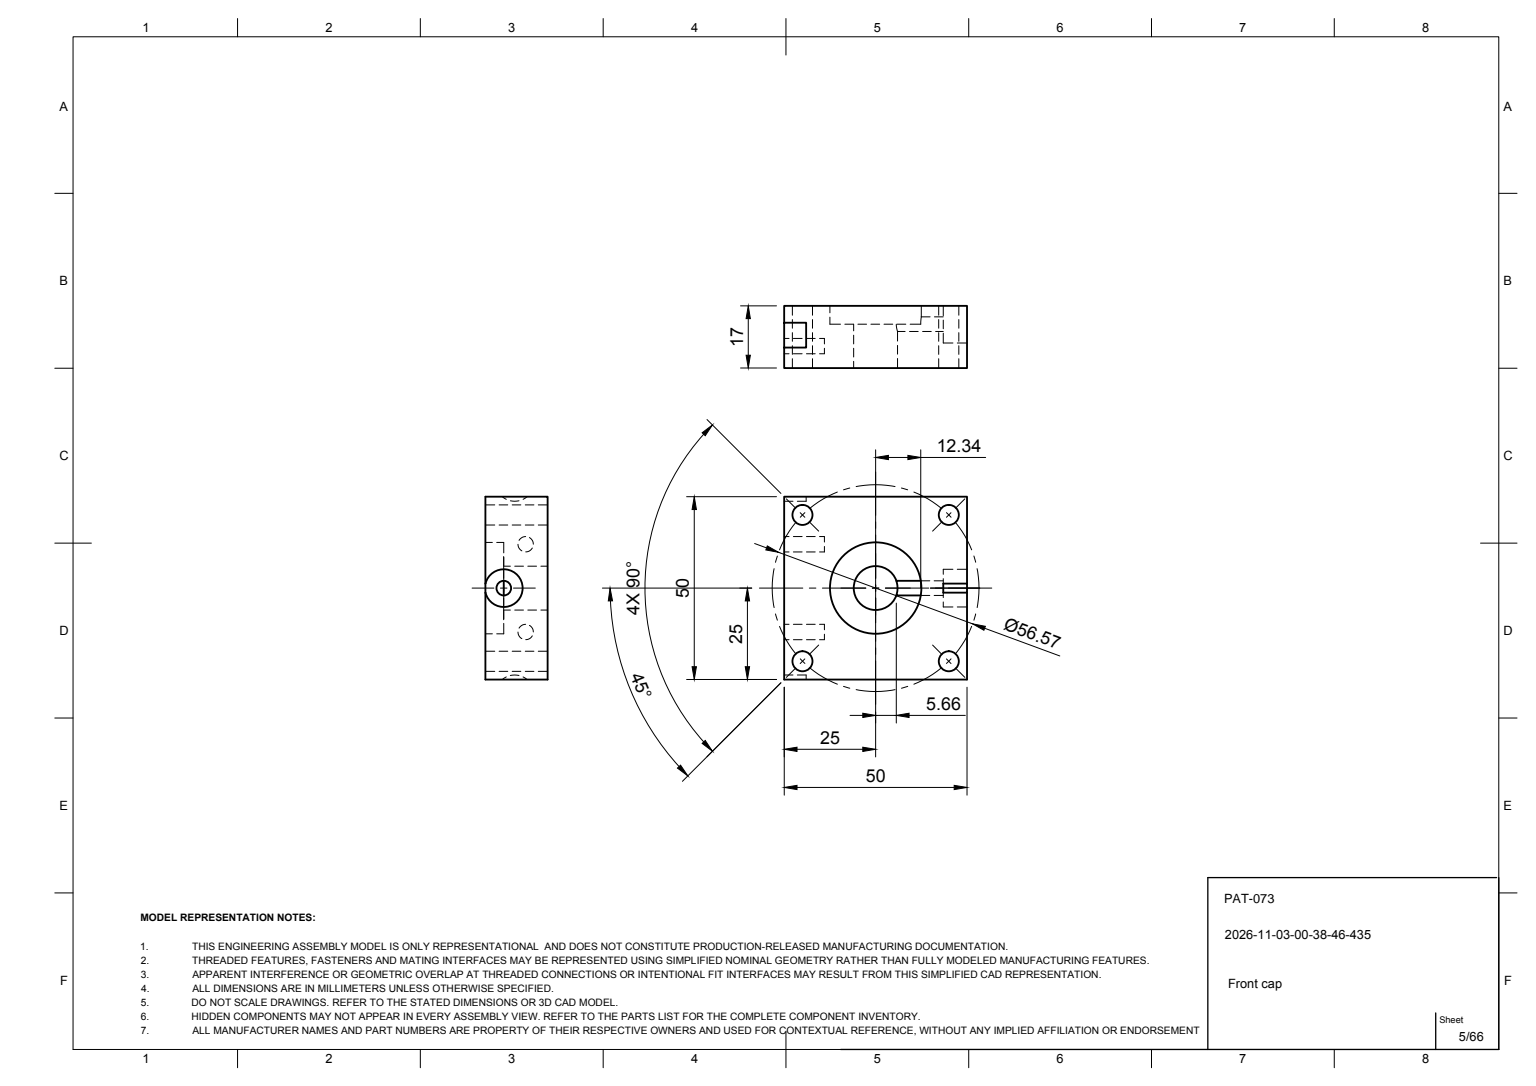
ISO-10303-21;
HEADER;
/* Generated by software containing ST-Developer
 * from STEP Tools, Inc. (www.steptools.com) 
 */

FILE_DESCRIPTION(
/* description */ ('Manual piston pump'),
/* implementation_level */ '2;1');

FILE_NAME(
/* name */ 'Front cap.step',
/* time_stamp */ '2026-11-02T16:54:23-08:00',
/* author */ (''),
/* organization */ (''),
/* preprocessor_version */ 'ST-DEVELOPER v20.2',
/* originating_system */ 'Autodesk Translation Framework v15.17.0.0',
/* authorisation */ '');

FILE_SCHEMA (('AUTOMOTIVE_DESIGN { 1 0 10303 214 3 1 1 }'));
ENDSEC;

DATA;
#10=MECHANICAL_DESIGN_GEOMETRIC_PRESENTATION_REPRESENTATION('',(#688),#19043);
#562=SHAPE_REPRESENTATION_RELATIONSHIP('SRR','None',#19308,#625);
#625=ADVANCED_BREP_SHAPE_REPRESENTATION('',(#760),#18975);
#688=STYLED_ITEM('',(#19661),#760);
#760=MANIFOLD_SOLID_BREP('Body1',#9472);
#827=FACE_BOUND('',#1879,.T.);
#828=FACE_BOUND('',#1882,.T.);
#829=FACE_BOUND('',#1883,.T.);
#830=FACE_BOUND('',#1884,.T.);
#831=FACE_BOUND('',#1885,.T.);
#832=FACE_BOUND('',#1886,.T.);
#833=FACE_BOUND('',#1895,.T.);
#834=FACE_BOUND('',#1896,.T.);
#835=FACE_BOUND('',#1897,.T.);
#836=FACE_BOUND('',#1898,.T.);
#837=FACE_BOUND('',#1899,.T.);
#838=FACE_BOUND('',#1902,.T.);
#839=FACE_BOUND('',#1903,.T.);
#1048=B_SPLINE_CURVE_WITH_KNOTS('',3,(#14655,#14656,#14657,#14658,#14659,
#14660,#14661,#14662,#14663,#14664,#14665,#14666,#14667,#14668,#14669,#14670,
#14671,#14672),.UNSPECIFIED.,.F.,.F.,(4,2,2,2,2,2,2,2,4),(0.,0.0754777383366878,
0.150955476673376,0.226431506332747,0.301907535992118,0.377383565651489,
0.45285959531086,0.528337333647548,0.603815071984236),.UNSPECIFIED.);
#1049=B_SPLINE_CURVE_WITH_KNOTS('',3,(#14676,#14677,#14678,#14679,#14680,
#14681,#14682,#14683,#14684,#14685,#14686,#14687,#14688,#14689,#14690,#14691,
#14692,#14693),.UNSPECIFIED.,.F.,.F.,(4,2,2,2,2,2,2,2,4),(-0.607760117460593,
-0.531772481215855,-0.455784844971118,-0.379832451850707,-0.303880058730296,
-0.227927665609885,-0.151975272489475,-0.0759876362447374,0.),
 .UNSPECIFIED.);
#1091=CYLINDRICAL_SURFACE('',#10248,0.525);
#1092=CYLINDRICAL_SURFACE('',#10250,0.525);
#1093=CYLINDRICAL_SURFACE('',#10255,0.21);
#1094=CYLINDRICAL_SURFACE('',#10259,0.21);
#1095=CYLINDRICAL_SURFACE('',#10263,0.2);
#1096=CYLINDRICAL_SURFACE('',#10265,0.6);
#1097=CYLINDRICAL_SURFACE('',#10271,0.515);
#1098=CYLINDRICAL_SURFACE('',#10279,0.275);
#1099=CYLINDRICAL_SURFACE('',#10281,0.275);
#1100=CYLINDRICAL_SURFACE('',#10283,0.275);
#1101=CYLINDRICAL_SURFACE('',#10285,0.275);
#1102=CYLINDRICAL_SURFACE('',#10287,1.25);
#1292=FACE_OUTER_BOUND('',#1867,.T.);
#1293=FACE_OUTER_BOUND('',#1868,.T.);
#1294=FACE_OUTER_BOUND('',#1869,.T.);
#1295=FACE_OUTER_BOUND('',#1870,.T.);
#1296=FACE_OUTER_BOUND('',#1871,.T.);
#1297=FACE_OUTER_BOUND('',#1872,.T.);
#1298=FACE_OUTER_BOUND('',#1873,.T.);
#1299=FACE_OUTER_BOUND('',#1874,.T.);
#1300=FACE_OUTER_BOUND('',#1875,.T.);
#1301=FACE_OUTER_BOUND('',#1876,.T.);
#1302=FACE_OUTER_BOUND('',#1877,.T.);
#1303=FACE_OUTER_BOUND('',#1878,.T.);
#1304=FACE_OUTER_BOUND('',#1880,.T.);
#1305=FACE_OUTER_BOUND('',#1881,.T.);
#1306=FACE_OUTER_BOUND('',#1887,.T.);
#1307=FACE_OUTER_BOUND('',#1888,.T.);
#1308=FACE_OUTER_BOUND('',#1889,.T.);
#1309=FACE_OUTER_BOUND('',#1890,.T.);
#1310=FACE_OUTER_BOUND('',#1891,.T.);
#1311=FACE_OUTER_BOUND('',#1892,.T.);
#1312=FACE_OUTER_BOUND('',#1893,.T.);
#1313=FACE_OUTER_BOUND('',#1894,.T.);
#1314=FACE_OUTER_BOUND('',#1900,.T.);
#1315=FACE_OUTER_BOUND('',#1901,.T.);
#1867=EDGE_LOOP('',(#6273,#6274));
#1868=EDGE_LOOP('',(#6275,#6276,#6277,#6278));
#1869=EDGE_LOOP('',(#6279,#6280,#6281,#6282));
#1870=EDGE_LOOP('',(#6283,#6284));
#1871=EDGE_LOOP('',(#6285,#6286,#6287,#6288,#6289,#6290,#6291,#6292));
#1872=EDGE_LOOP('',(#6293,#6294,#6295,#6296));
#1873=EDGE_LOOP('',(#6297));
#1874=EDGE_LOOP('',(#6298,#6299,#6300,#6301));
#1875=EDGE_LOOP('',(#6302));
#1876=EDGE_LOOP('',(#6303,#6304,#6305,#6306,#6307,#6308,#6309));
#1877=EDGE_LOOP('',(#6310,#6311,#6312,#6313,#6314,#6315));
#1878=EDGE_LOOP('',(#6316,#6317));
#1879=EDGE_LOOP('',(#6318));
#1880=EDGE_LOOP('',(#6319,#6320,#6321,#6322));
#1881=EDGE_LOOP('',(#6323,#6324,#6325,#6326,#6327,#6328,#6329,#6330));
#1882=EDGE_LOOP('',(#6331));
#1883=EDGE_LOOP('',(#6332));
#1884=EDGE_LOOP('',(#6333));
#1885=EDGE_LOOP('',(#6334));
#1886=EDGE_LOOP('',(#6335));
#1887=EDGE_LOOP('',(#6336,#6337,#6338,#6339));
#1888=EDGE_LOOP('',(#6340,#6341,#6342,#6343));
#1889=EDGE_LOOP('',(#6344,#6345,#6346,#6347));
#1890=EDGE_LOOP('',(#6348,#6349,#6350,#6351));
#1891=EDGE_LOOP('',(#6352,#6353,#6354,#6355,#6356,#6357));
#1892=EDGE_LOOP('',(#6358,#6359,#6360,#6361,#6362,#6363));
#1893=EDGE_LOOP('',(#6364,#6365,#6366,#6367,#6368,#6369,#6370,#6371));
#1894=EDGE_LOOP('',(#6372,#6373,#6374,#6375));
#1895=EDGE_LOOP('',(#6376));
#1896=EDGE_LOOP('',(#6377));
#1897=EDGE_LOOP('',(#6378));
#1898=EDGE_LOOP('',(#6379));
#1899=EDGE_LOOP('',(#6380));
#1900=EDGE_LOOP('',(#6381,#6382,#6383,#6384,#6385,#6386));
#1901=EDGE_LOOP('',(#6387,#6388,#6389,#6390,#6391,#6392,#6393,#6394));
#1902=EDGE_LOOP('',(#6395));
#1903=EDGE_LOOP('',(#6396));
#2663=CIRCLE('',#10247,0.525);
#2664=CIRCLE('',#10249,0.525);
#2665=CIRCLE('',#10251,0.525);
#2666=CIRCLE('',#10252,0.525);
#2667=CIRCLE('',#10256,0.21);
#2668=CIRCLE('',#10257,0.21);
#2669=CIRCLE('',#10260,0.21);
#2670=CIRCLE('',#10261,0.21);
#2671=CIRCLE('',#10264,0.2);
#2672=CIRCLE('',#10266,0.6);
#2673=CIRCLE('',#10267,0.6);
#2674=CIRCLE('',#10268,0.6);
#2675=CIRCLE('',#10270,0.515);
#2676=CIRCLE('',#10272,0.515);
#2677=CIRCLE('',#10274,0.275);
#2678=CIRCLE('',#10275,0.275);
#2679=CIRCLE('',#10276,0.275);
#2680=CIRCLE('',#10277,0.275);
#2681=CIRCLE('',#10278,1.25);
#2682=CIRCLE('',#10280,0.275);
#2683=CIRCLE('',#10282,0.275);
#2684=CIRCLE('',#10284,0.275);
#2685=CIRCLE('',#10286,0.275);
#2686=CIRCLE('',#10288,1.25);
#2687=CIRCLE('',#10289,1.25);
#3147=LINE('',#14609,#3751);
#3148=LINE('',#14613,#3752);
#3149=LINE('',#14616,#3753);
#3150=LINE('',#14620,#3754);
#3151=LINE('',#14624,#3755);
#3152=LINE('',#14627,#3756);
#3153=LINE('',#14630,#3757);
#3154=LINE('',#14632,#3758);
#3155=LINE('',#14634,#3759);
#3156=LINE('',#14636,#3760);
#3157=LINE('',#14637,#3761);
#3158=LINE('',#14642,#3762);
#3159=LINE('',#14649,#3763);
#3160=LINE('',#14674,#3764);
#3161=LINE('',#14694,#3765);
#3162=LINE('',#14696,#3766);
#3163=LINE('',#14702,#3767);
#3164=LINE('',#14708,#3768);
#3165=LINE('',#14712,#3769);
#3166=LINE('',#14715,#3770);
#3167=LINE('',#14718,#3771);
#3168=LINE('',#14720,#3772);
#3169=LINE('',#14721,#3773);
#3170=LINE('',#14722,#3774);
#3171=LINE('',#14736,#3775);
#3172=LINE('',#14740,#3776);
#3173=LINE('',#14744,#3777);
#3174=LINE('',#14748,#3778);
#3175=LINE('',#14752,#3779);
#3176=LINE('',#14756,#3780);
#3177=LINE('',#14758,#3781);
#3178=LINE('',#14760,#3782);
#3179=LINE('',#14761,#3783);
#3180=LINE('',#14763,#3784);
#3181=LINE('',#14764,#3785);
#3751=VECTOR('',#11503,1.);
#3752=VECTOR('',#11508,1.);
#3753=VECTOR('',#11511,1.);
#3754=VECTOR('',#11514,1.);
#3755=VECTOR('',#11517,1.);
#3756=VECTOR('',#11522,1.);
#3757=VECTOR('',#11525,1.);
#3758=VECTOR('',#11526,1.);
#3759=VECTOR('',#11527,1.);
#3760=VECTOR('',#11528,1.);
#3761=VECTOR('',#11529,1.);
#3762=VECTOR('',#11534,0.21);
#3763=VECTOR('',#11543,0.21);
#3764=VECTOR('',#11550,1.);
#3765=VECTOR('',#11551,1.);
#3766=VECTOR('',#11552,0.2);
#3767=VECTOR('',#11559,0.6);
#3768=VECTOR('',#11566,1.);
#3769=VECTOR('',#11571,1.);
#3770=VECTOR('',#11574,1.);
#3771=VECTOR('',#11577,1.);
#3772=VECTOR('',#11578,1.);
#3773=VECTOR('',#11579,1.);
#3774=VECTOR('',#11580,1.);
#3775=VECTOR('',#11595,0.275);
#3776=VECTOR('',#11600,0.275);
#3777=VECTOR('',#11605,0.275);
#3778=VECTOR('',#11610,0.275);
#3779=VECTOR('',#11615,1.25);
#3780=VECTOR('',#11622,1.);
#3781=VECTOR('',#11623,1.);
#3782=VECTOR('',#11624,1.);
#3783=VECTOR('',#11625,1.);
#3784=VECTOR('',#11628,1.);
#3785=VECTOR('',#11629,1.);
#4355=VERTEX_POINT('',#14607);
#4356=VERTEX_POINT('',#14608);
#4357=VERTEX_POINT('',#14612);
#4358=VERTEX_POINT('',#14614);
#4359=VERTEX_POINT('',#14618);
#4360=VERTEX_POINT('',#14619);
#4361=VERTEX_POINT('',#14621);
#4362=VERTEX_POINT('',#14623);
#4363=VERTEX_POINT('',#14629);
#4364=VERTEX_POINT('',#14631);
#4365=VERTEX_POINT('',#14633);
#4366=VERTEX_POINT('',#14635);
#4367=VERTEX_POINT('',#14639);
#4368=VERTEX_POINT('',#14641);
#4369=VERTEX_POINT('',#14646);
#4370=VERTEX_POINT('',#14648);
#4371=VERTEX_POINT('',#14653);
#4372=VERTEX_POINT('',#14654);
#4373=VERTEX_POINT('',#14673);
#4374=VERTEX_POINT('',#14675);
#4375=VERTEX_POINT('',#14695);
#4376=VERTEX_POINT('',#14699);
#4377=VERTEX_POINT('',#14701);
#4378=VERTEX_POINT('',#14706);
#4379=VERTEX_POINT('',#14707);
#4380=VERTEX_POINT('',#14711);
#4381=VERTEX_POINT('',#14713);
#4382=VERTEX_POINT('',#14717);
#4383=VERTEX_POINT('',#14719);
#4384=VERTEX_POINT('',#14723);
#4385=VERTEX_POINT('',#14725);
#4386=VERTEX_POINT('',#14727);
#4387=VERTEX_POINT('',#14729);
#4388=VERTEX_POINT('',#14731);
#4389=VERTEX_POINT('',#14734);
#4390=VERTEX_POINT('',#14738);
#4391=VERTEX_POINT('',#14742);
#4392=VERTEX_POINT('',#14746);
#4393=VERTEX_POINT('',#14750);
#4394=VERTEX_POINT('',#14757);
#4395=VERTEX_POINT('',#14759);
#5123=EDGE_CURVE('',#4355,#4356,#3147,.T.);
#5124=EDGE_CURVE('',#4356,#4355,#2663,.T.);
#5125=EDGE_CURVE('',#4357,#4355,#3148,.T.);
#5126=EDGE_CURVE('',#4358,#4357,#2664,.T.);
#5127=EDGE_CURVE('',#4356,#4358,#3149,.T.);
#5128=EDGE_CURVE('',#4359,#4360,#3150,.T.);
#5129=EDGE_CURVE('',#4359,#4361,#2665,.T.);
#5130=EDGE_CURVE('',#4362,#4361,#3151,.T.);
#5131=EDGE_CURVE('',#4360,#4362,#2666,.T.);
#5132=EDGE_CURVE('',#4361,#4359,#3152,.T.);
#5133=EDGE_CURVE('',#4358,#4363,#3153,.T.);
#5134=EDGE_CURVE('',#4363,#4364,#3154,.T.);
#5135=EDGE_CURVE('',#4365,#4364,#3155,.T.);
#5136=EDGE_CURVE('',#4366,#4365,#3156,.T.);
#5137=EDGE_CURVE('',#4366,#4357,#3157,.T.);
#5138=EDGE_CURVE('',#4367,#4367,#2667,.T.);
#5139=EDGE_CURVE('',#4367,#4368,#3158,.T.);
#5140=EDGE_CURVE('',#4368,#4368,#2668,.T.);
#5141=EDGE_CURVE('',#4369,#4369,#2669,.T.);
#5142=EDGE_CURVE('',#4369,#4370,#3159,.T.);
#5143=EDGE_CURVE('',#4370,#4370,#2670,.T.);
#5144=EDGE_CURVE('',#4371,#4372,#1048,.T.);
#5145=EDGE_CURVE('',#4373,#4371,#3160,.T.);
#5146=EDGE_CURVE('',#4374,#4373,#1049,.T.);
#5147=EDGE_CURVE('',#4372,#4374,#3161,.T.);
#5148=EDGE_CURVE('',#4372,#4375,#3162,.T.);
#5149=EDGE_CURVE('',#4375,#4375,#2671,.T.);
#5150=EDGE_CURVE('',#4376,#4376,#2672,.T.);
#5151=EDGE_CURVE('',#4376,#4377,#3163,.T.);
#5152=EDGE_CURVE('',#4374,#4377,#2673,.T.);
#5153=EDGE_CURVE('',#4377,#4373,#2674,.T.);
#5154=EDGE_CURVE('',#4378,#4379,#3164,.T.);
#5155=EDGE_CURVE('',#4378,#4379,#2675,.T.);
#5156=EDGE_CURVE('',#4380,#4378,#3165,.T.);
#5157=EDGE_CURVE('',#4381,#4380,#2676,.T.);
#5158=EDGE_CURVE('',#4379,#4381,#3166,.T.);
#5159=EDGE_CURVE('',#4382,#4381,#3167,.T.);
#5160=EDGE_CURVE('',#4383,#4382,#3168,.T.);
#5161=EDGE_CURVE('',#4383,#4366,#3169,.T.);
#5162=EDGE_CURVE('',#4380,#4365,#3170,.T.);
#5163=EDGE_CURVE('',#4384,#4384,#2677,.T.);
#5164=EDGE_CURVE('',#4385,#4385,#2678,.T.);
#5165=EDGE_CURVE('',#4386,#4386,#2679,.T.);
#5166=EDGE_CURVE('',#4387,#4387,#2680,.T.);
#5167=EDGE_CURVE('',#4388,#4388,#2681,.T.);
#5168=EDGE_CURVE('',#4389,#4389,#2682,.T.);
#5169=EDGE_CURVE('',#4389,#4384,#3171,.T.);
#5170=EDGE_CURVE('',#4390,#4390,#2683,.T.);
#5171=EDGE_CURVE('',#4390,#4385,#3172,.T.);
#5172=EDGE_CURVE('',#4391,#4391,#2684,.T.);
#5173=EDGE_CURVE('',#4391,#4386,#3173,.T.);
#5174=EDGE_CURVE('',#4392,#4392,#2685,.T.);
#5175=EDGE_CURVE('',#4392,#4387,#3174,.T.);
#5176=EDGE_CURVE('',#4393,#4372,#2686,.T.);
#5177=EDGE_CURVE('',#4393,#4388,#3175,.T.);
#5178=EDGE_CURVE('',#4371,#4393,#2687,.T.);
#5179=EDGE_CURVE('',#4360,#4383,#3176,.T.);
#5180=EDGE_CURVE('',#4394,#4382,#3177,.T.);
#5181=EDGE_CURVE('',#4395,#4394,#3178,.T.);
#5182=EDGE_CURVE('',#4395,#4362,#3179,.T.);
#5183=EDGE_CURVE('',#4363,#4395,#3180,.T.);
#5184=EDGE_CURVE('',#4364,#4394,#3181,.T.);
#6273=ORIENTED_EDGE('',*,*,#5123,.F.);
#6274=ORIENTED_EDGE('',*,*,#5124,.F.);
#6275=ORIENTED_EDGE('',*,*,#5125,.F.);
#6276=ORIENTED_EDGE('',*,*,#5126,.F.);
#6277=ORIENTED_EDGE('',*,*,#5127,.F.);
#6278=ORIENTED_EDGE('',*,*,#5124,.T.);
#6279=ORIENTED_EDGE('',*,*,#5128,.F.);
#6280=ORIENTED_EDGE('',*,*,#5129,.T.);
#6281=ORIENTED_EDGE('',*,*,#5130,.F.);
#6282=ORIENTED_EDGE('',*,*,#5131,.F.);
#6283=ORIENTED_EDGE('',*,*,#5132,.F.);
#6284=ORIENTED_EDGE('',*,*,#5129,.F.);
#6285=ORIENTED_EDGE('',*,*,#5125,.T.);
#6286=ORIENTED_EDGE('',*,*,#5123,.T.);
#6287=ORIENTED_EDGE('',*,*,#5127,.T.);
#6288=ORIENTED_EDGE('',*,*,#5133,.T.);
#6289=ORIENTED_EDGE('',*,*,#5134,.T.);
#6290=ORIENTED_EDGE('',*,*,#5135,.F.);
#6291=ORIENTED_EDGE('',*,*,#5136,.F.);
#6292=ORIENTED_EDGE('',*,*,#5137,.T.);
#6293=ORIENTED_EDGE('',*,*,#5138,.F.);
#6294=ORIENTED_EDGE('',*,*,#5139,.T.);
#6295=ORIENTED_EDGE('',*,*,#5140,.T.);
#6296=ORIENTED_EDGE('',*,*,#5139,.F.);
#6297=ORIENTED_EDGE('',*,*,#5140,.F.);
#6298=ORIENTED_EDGE('',*,*,#5141,.F.);
#6299=ORIENTED_EDGE('',*,*,#5142,.T.);
#6300=ORIENTED_EDGE('',*,*,#5143,.T.);
#6301=ORIENTED_EDGE('',*,*,#5142,.F.);
#6302=ORIENTED_EDGE('',*,*,#5143,.F.);
#6303=ORIENTED_EDGE('',*,*,#5144,.F.);
#6304=ORIENTED_EDGE('',*,*,#5145,.F.);
#6305=ORIENTED_EDGE('',*,*,#5146,.F.);
#6306=ORIENTED_EDGE('',*,*,#5147,.F.);
#6307=ORIENTED_EDGE('',*,*,#5148,.T.);
#6308=ORIENTED_EDGE('',*,*,#5149,.F.);
#6309=ORIENTED_EDGE('',*,*,#5148,.F.);
#6310=ORIENTED_EDGE('',*,*,#5150,.F.);
#6311=ORIENTED_EDGE('',*,*,#5151,.T.);
#6312=ORIENTED_EDGE('',*,*,#5152,.F.);
#6313=ORIENTED_EDGE('',*,*,#5146,.T.);
#6314=ORIENTED_EDGE('',*,*,#5153,.F.);
#6315=ORIENTED_EDGE('',*,*,#5151,.F.);
#6316=ORIENTED_EDGE('',*,*,#5154,.F.);
#6317=ORIENTED_EDGE('',*,*,#5155,.T.);
#6318=ORIENTED_EDGE('',*,*,#5149,.T.);
#6319=ORIENTED_EDGE('',*,*,#5156,.F.);
#6320=ORIENTED_EDGE('',*,*,#5157,.F.);
#6321=ORIENTED_EDGE('',*,*,#5158,.F.);
#6322=ORIENTED_EDGE('',*,*,#5155,.F.);
#6323=ORIENTED_EDGE('',*,*,#5156,.T.);
#6324=ORIENTED_EDGE('',*,*,#5154,.T.);
#6325=ORIENTED_EDGE('',*,*,#5158,.T.);
#6326=ORIENTED_EDGE('',*,*,#5159,.F.);
#6327=ORIENTED_EDGE('',*,*,#5160,.F.);
#6328=ORIENTED_EDGE('',*,*,#5161,.T.);
#6329=ORIENTED_EDGE('',*,*,#5136,.T.);
#6330=ORIENTED_EDGE('',*,*,#5162,.F.);
#6331=ORIENTED_EDGE('',*,*,#5163,.T.);
#6332=ORIENTED_EDGE('',*,*,#5164,.T.);
#6333=ORIENTED_EDGE('',*,*,#5165,.T.);
#6334=ORIENTED_EDGE('',*,*,#5166,.T.);
#6335=ORIENTED_EDGE('',*,*,#5167,.T.);
#6336=ORIENTED_EDGE('',*,*,#5168,.F.);
#6337=ORIENTED_EDGE('',*,*,#5169,.T.);
#6338=ORIENTED_EDGE('',*,*,#5163,.F.);
#6339=ORIENTED_EDGE('',*,*,#5169,.F.);
#6340=ORIENTED_EDGE('',*,*,#5170,.F.);
#6341=ORIENTED_EDGE('',*,*,#5171,.T.);
#6342=ORIENTED_EDGE('',*,*,#5164,.F.);
#6343=ORIENTED_EDGE('',*,*,#5171,.F.);
#6344=ORIENTED_EDGE('',*,*,#5172,.F.);
#6345=ORIENTED_EDGE('',*,*,#5173,.T.);
#6346=ORIENTED_EDGE('',*,*,#5165,.F.);
#6347=ORIENTED_EDGE('',*,*,#5173,.F.);
#6348=ORIENTED_EDGE('',*,*,#5174,.F.);
#6349=ORIENTED_EDGE('',*,*,#5175,.T.);
#6350=ORIENTED_EDGE('',*,*,#5166,.F.);
#6351=ORIENTED_EDGE('',*,*,#5175,.F.);
#6352=ORIENTED_EDGE('',*,*,#5144,.T.);
#6353=ORIENTED_EDGE('',*,*,#5176,.F.);
#6354=ORIENTED_EDGE('',*,*,#5177,.T.);
#6355=ORIENTED_EDGE('',*,*,#5167,.F.);
#6356=ORIENTED_EDGE('',*,*,#5177,.F.);
#6357=ORIENTED_EDGE('',*,*,#5178,.F.);
#6358=ORIENTED_EDGE('',*,*,#5147,.T.);
#6359=ORIENTED_EDGE('',*,*,#5152,.T.);
#6360=ORIENTED_EDGE('',*,*,#5153,.T.);
#6361=ORIENTED_EDGE('',*,*,#5145,.T.);
#6362=ORIENTED_EDGE('',*,*,#5178,.T.);
#6363=ORIENTED_EDGE('',*,*,#5176,.T.);
#6364=ORIENTED_EDGE('',*,*,#5128,.T.);
#6365=ORIENTED_EDGE('',*,*,#5179,.T.);
#6366=ORIENTED_EDGE('',*,*,#5160,.T.);
#6367=ORIENTED_EDGE('',*,*,#5180,.F.);
#6368=ORIENTED_EDGE('',*,*,#5181,.F.);
#6369=ORIENTED_EDGE('',*,*,#5182,.T.);
#6370=ORIENTED_EDGE('',*,*,#5130,.T.);
#6371=ORIENTED_EDGE('',*,*,#5132,.T.);
#6372=ORIENTED_EDGE('',*,*,#5183,.T.);
#6373=ORIENTED_EDGE('',*,*,#5181,.T.);
#6374=ORIENTED_EDGE('',*,*,#5184,.F.);
#6375=ORIENTED_EDGE('',*,*,#5134,.F.);
#6376=ORIENTED_EDGE('',*,*,#5150,.T.);
#6377=ORIENTED_EDGE('',*,*,#5174,.T.);
#6378=ORIENTED_EDGE('',*,*,#5172,.T.);
#6379=ORIENTED_EDGE('',*,*,#5170,.T.);
#6380=ORIENTED_EDGE('',*,*,#5168,.T.);
#6381=ORIENTED_EDGE('',*,*,#5157,.T.);
#6382=ORIENTED_EDGE('',*,*,#5162,.T.);
#6383=ORIENTED_EDGE('',*,*,#5135,.T.);
#6384=ORIENTED_EDGE('',*,*,#5184,.T.);
#6385=ORIENTED_EDGE('',*,*,#5180,.T.);
#6386=ORIENTED_EDGE('',*,*,#5159,.T.);
#6387=ORIENTED_EDGE('',*,*,#5126,.T.);
#6388=ORIENTED_EDGE('',*,*,#5137,.F.);
#6389=ORIENTED_EDGE('',*,*,#5161,.F.);
#6390=ORIENTED_EDGE('',*,*,#5179,.F.);
#6391=ORIENTED_EDGE('',*,*,#5131,.T.);
#6392=ORIENTED_EDGE('',*,*,#5182,.F.);
#6393=ORIENTED_EDGE('',*,*,#5183,.F.);
#6394=ORIENTED_EDGE('',*,*,#5133,.F.);
#6395=ORIENTED_EDGE('',*,*,#5138,.T.);
#6396=ORIENTED_EDGE('',*,*,#5141,.T.);
#8573=PLANE('',#10246);
#8574=PLANE('',#10253);
#8575=PLANE('',#10254);
#8576=PLANE('',#10258);
#8577=PLANE('',#10262);
#8578=PLANE('',#10269);
#8579=PLANE('',#10273);
#8580=PLANE('',#10290);
#8581=PLANE('',#10291);
#8582=PLANE('',#10292);
#8583=PLANE('',#10293);
#8584=PLANE('',#10294);
#8897=ADVANCED_FACE('',(#1292),#8573,.F.);
#8898=ADVANCED_FACE('',(#1293),#1091,.F.);
#8899=ADVANCED_FACE('',(#1294),#1092,.F.);
#8900=ADVANCED_FACE('',(#1295),#8574,.F.);
#8901=ADVANCED_FACE('',(#1296),#8575,.T.);
#8902=ADVANCED_FACE('',(#1297),#1093,.F.);
#8903=ADVANCED_FACE('',(#1298),#8576,.F.);
#8904=ADVANCED_FACE('',(#1299),#1094,.F.);
#8905=ADVANCED_FACE('',(#1300),#8577,.F.);
#8906=ADVANCED_FACE('',(#1301),#1095,.F.);
#8907=ADVANCED_FACE('',(#1302),#1096,.F.);
#8908=ADVANCED_FACE('',(#1303,#827),#8578,.T.);
#8909=ADVANCED_FACE('',(#1304),#1097,.F.);
#8910=ADVANCED_FACE('',(#1305,#828,#829,#830,#831,#832),#8579,.T.);
#8911=ADVANCED_FACE('',(#1306),#1098,.F.);
#8912=ADVANCED_FACE('',(#1307),#1099,.F.);
#8913=ADVANCED_FACE('',(#1308),#1100,.F.);
#8914=ADVANCED_FACE('',(#1309),#1101,.F.);
#8915=ADVANCED_FACE('',(#1310),#1102,.F.);
#8916=ADVANCED_FACE('',(#1311),#8580,.T.);
#8917=ADVANCED_FACE('',(#1312),#8581,.T.);
#8918=ADVANCED_FACE('',(#1313,#833,#834,#835,#836,#837),#8582,.T.);
#8919=ADVANCED_FACE('',(#1314),#8583,.T.);
#8920=ADVANCED_FACE('',(#1315,#838,#839),#8584,.F.);
#9472=CLOSED_SHELL('',(#8897,#8898,#8899,#8900,#8901,#8902,#8903,#8904,
#8905,#8906,#8907,#8908,#8909,#8910,#8911,#8912,#8913,#8914,#8915,#8916,
#8917,#8918,#8919,#8920));
#10245=AXIS2_PLACEMENT_3D('',#14605,#11499,#11500);
#10246=AXIS2_PLACEMENT_3D('',#14606,#11501,#11502);
#10247=AXIS2_PLACEMENT_3D('',#14610,#11504,#11505);
#10248=AXIS2_PLACEMENT_3D('',#14611,#11506,#11507);
#10249=AXIS2_PLACEMENT_3D('',#14615,#11509,#11510);
#10250=AXIS2_PLACEMENT_3D('',#14617,#11512,#11513);
#10251=AXIS2_PLACEMENT_3D('',#14622,#11515,#11516);
#10252=AXIS2_PLACEMENT_3D('',#14625,#11518,#11519);
#10253=AXIS2_PLACEMENT_3D('',#14626,#11520,#11521);
#10254=AXIS2_PLACEMENT_3D('',#14628,#11523,#11524);
#10255=AXIS2_PLACEMENT_3D('',#14638,#11530,#11531);
#10256=AXIS2_PLACEMENT_3D('',#14640,#11532,#11533);
#10257=AXIS2_PLACEMENT_3D('',#14643,#11535,#11536);
#10258=AXIS2_PLACEMENT_3D('',#14644,#11537,#11538);
#10259=AXIS2_PLACEMENT_3D('',#14645,#11539,#11540);
#10260=AXIS2_PLACEMENT_3D('',#14647,#11541,#11542);
#10261=AXIS2_PLACEMENT_3D('',#14650,#11544,#11545);
#10262=AXIS2_PLACEMENT_3D('',#14651,#11546,#11547);
#10263=AXIS2_PLACEMENT_3D('',#14652,#11548,#11549);
#10264=AXIS2_PLACEMENT_3D('',#14697,#11553,#11554);
#10265=AXIS2_PLACEMENT_3D('',#14698,#11555,#11556);
#10266=AXIS2_PLACEMENT_3D('',#14700,#11557,#11558);
#10267=AXIS2_PLACEMENT_3D('',#14703,#11560,#11561);
#10268=AXIS2_PLACEMENT_3D('',#14704,#11562,#11563);
#10269=AXIS2_PLACEMENT_3D('',#14705,#11564,#11565);
#10270=AXIS2_PLACEMENT_3D('',#14709,#11567,#11568);
#10271=AXIS2_PLACEMENT_3D('',#14710,#11569,#11570);
#10272=AXIS2_PLACEMENT_3D('',#14714,#11572,#11573);
#10273=AXIS2_PLACEMENT_3D('',#14716,#11575,#11576);
#10274=AXIS2_PLACEMENT_3D('',#14724,#11581,#11582);
#10275=AXIS2_PLACEMENT_3D('',#14726,#11583,#11584);
#10276=AXIS2_PLACEMENT_3D('',#14728,#11585,#11586);
#10277=AXIS2_PLACEMENT_3D('',#14730,#11587,#11588);
#10278=AXIS2_PLACEMENT_3D('',#14732,#11589,#11590);
#10279=AXIS2_PLACEMENT_3D('',#14733,#11591,#11592);
#10280=AXIS2_PLACEMENT_3D('',#14735,#11593,#11594);
#10281=AXIS2_PLACEMENT_3D('',#14737,#11596,#11597);
#10282=AXIS2_PLACEMENT_3D('',#14739,#11598,#11599);
#10283=AXIS2_PLACEMENT_3D('',#14741,#11601,#11602);
#10284=AXIS2_PLACEMENT_3D('',#14743,#11603,#11604);
#10285=AXIS2_PLACEMENT_3D('',#14745,#11606,#11607);
#10286=AXIS2_PLACEMENT_3D('',#14747,#11608,#11609);
#10287=AXIS2_PLACEMENT_3D('',#14749,#11611,#11612);
#10288=AXIS2_PLACEMENT_3D('',#14751,#11613,#11614);
#10289=AXIS2_PLACEMENT_3D('',#14753,#11616,#11617);
#10290=AXIS2_PLACEMENT_3D('',#14754,#11618,#11619);
#10291=AXIS2_PLACEMENT_3D('',#14755,#11620,#11621);
#10292=AXIS2_PLACEMENT_3D('',#14762,#11626,#11627);
#10293=AXIS2_PLACEMENT_3D('',#14765,#11630,#11631);
#10294=AXIS2_PLACEMENT_3D('',#14766,#11632,#11633);
#11499=DIRECTION('axis',(0.,0.,1.));
#11500=DIRECTION('refdir',(1.,0.,0.));
#11501=DIRECTION('center_axis',(0.,0.,1.));
#11502=DIRECTION('ref_axis',(1.,0.,0.));
#11503=DIRECTION('',(0.,-1.,0.));
#11504=DIRECTION('center_axis',(0.,0.,1.));
#11505=DIRECTION('ref_axis',(1.,0.,0.));
#11506=DIRECTION('center_axis',(0.,0.,1.));
#11507=DIRECTION('ref_axis',(1.,0.,0.));
#11508=DIRECTION('',(0.,0.,1.));
#11509=DIRECTION('center_axis',(0.,0.,1.));
#11510=DIRECTION('ref_axis',(1.,0.,0.));
#11511=DIRECTION('',(0.,0.,-1.));
#11512=DIRECTION('center_axis',(0.,0.,1.));
#11513=DIRECTION('ref_axis',(-1.,1.22464679914735E-16,0.));
#11514=DIRECTION('',(0.,0.,-1.));
#11515=DIRECTION('center_axis',(0.,0.,1.));
#11516=DIRECTION('ref_axis',(1.,0.,0.));
#11517=DIRECTION('',(0.,0.,1.));
#11518=DIRECTION('center_axis',(0.,0.,1.));
#11519=DIRECTION('ref_axis',(1.,0.,0.));
#11520=DIRECTION('center_axis',(0.,0.,1.));
#11521=DIRECTION('ref_axis',(1.,0.,0.));
#11522=DIRECTION('',(0.,1.,0.));
#11523=DIRECTION('center_axis',(-1.,0.,0.));
#11524=DIRECTION('ref_axis',(0.,-1.,0.));
#11525=DIRECTION('',(0.,-1.,0.));
#11526=DIRECTION('',(0.,0.,1.));
#11527=DIRECTION('',(0.,-1.,0.));
#11528=DIRECTION('',(0.,0.,1.));
#11529=DIRECTION('',(0.,-1.,0.));
#11530=DIRECTION('center_axis',(0.,0.,1.));
#11531=DIRECTION('ref_axis',(1.,0.,0.));
#11532=DIRECTION('center_axis',(0.,0.,1.));
#11533=DIRECTION('ref_axis',(1.,0.,0.));
#11534=DIRECTION('',(0.,0.,1.));
#11535=DIRECTION('center_axis',(0.,0.,1.));
#11536=DIRECTION('ref_axis',(1.,0.,0.));
#11537=DIRECTION('center_axis',(0.,0.,1.));
#11538=DIRECTION('ref_axis',(1.,0.,0.));
#11539=DIRECTION('center_axis',(0.,0.,1.));
#11540=DIRECTION('ref_axis',(1.,0.,0.));
#11541=DIRECTION('center_axis',(0.,0.,1.));
#11542=DIRECTION('ref_axis',(1.,0.,0.));
#11543=DIRECTION('',(0.,0.,1.));
#11544=DIRECTION('center_axis',(0.,0.,1.));
#11545=DIRECTION('ref_axis',(1.,0.,0.));
#11546=DIRECTION('center_axis',(0.,0.,1.));
#11547=DIRECTION('ref_axis',(1.,0.,0.));
#11548=DIRECTION('center_axis',(0.,0.,1.));
#11549=DIRECTION('ref_axis',(1.,0.,0.));
#11550=DIRECTION('',(0.,0.,1.));
#11551=DIRECTION('',(0.,0.,-1.));
#11552=DIRECTION('',(0.,0.,1.));
#11553=DIRECTION('center_axis',(0.,0.,-1.));
#11554=DIRECTION('ref_axis',(1.,0.,0.));
#11555=DIRECTION('center_axis',(0.,1.,0.));
#11556=DIRECTION('ref_axis',(1.,0.,0.));
#11557=DIRECTION('center_axis',(0.,1.,0.));
#11558=DIRECTION('ref_axis',(1.,0.,0.));
#11559=DIRECTION('',(0.,1.,0.));
#11560=DIRECTION('center_axis',(0.,-1.,0.));
#11561=DIRECTION('ref_axis',(1.,0.,0.));
#11562=DIRECTION('center_axis',(0.,-1.,0.));
#11563=DIRECTION('ref_axis',(1.,0.,0.));
#11564=DIRECTION('center_axis',(0.,0.,1.));
#11565=DIRECTION('ref_axis',(1.,0.,0.));
#11566=DIRECTION('',(1.,0.,0.));
#11567=DIRECTION('center_axis',(0.,0.,1.));
#11568=DIRECTION('ref_axis',(1.,0.,0.));
#11569=DIRECTION('center_axis',(0.,0.,1.));
#11570=DIRECTION('ref_axis',(-1.83697019872103E-16,-1.,0.));
#11571=DIRECTION('',(0.,0.,-1.));
#11572=DIRECTION('center_axis',(0.,0.,-1.));
#11573=DIRECTION('ref_axis',(1.,0.,0.));
#11574=DIRECTION('',(0.,0.,1.));
#11575=DIRECTION('center_axis',(0.,1.,0.));
#11576=DIRECTION('ref_axis',(-1.,0.,0.));
#11577=DIRECTION('',(-1.,0.,0.));
#11578=DIRECTION('',(0.,0.,1.));
#11579=DIRECTION('',(-1.,0.,0.));
#11580=DIRECTION('',(-1.,0.,0.));
#11581=DIRECTION('center_axis',(0.,-1.,0.));
#11582=DIRECTION('ref_axis',(1.,0.,0.));
#11583=DIRECTION('center_axis',(0.,-1.,0.));
#11584=DIRECTION('ref_axis',(1.,0.,0.));
#11585=DIRECTION('center_axis',(0.,-1.,0.));
#11586=DIRECTION('ref_axis',(1.,0.,0.));
#11587=DIRECTION('center_axis',(0.,-1.,0.));
#11588=DIRECTION('ref_axis',(1.,0.,0.));
#11589=DIRECTION('center_axis',(0.,-1.,0.));
#11590=DIRECTION('ref_axis',(1.,0.,0.));
#11591=DIRECTION('center_axis',(0.,1.,0.));
#11592=DIRECTION('ref_axis',(1.,0.,0.));
#11593=DIRECTION('center_axis',(0.,1.,0.));
#11594=DIRECTION('ref_axis',(1.,0.,0.));
#11595=DIRECTION('',(0.,1.,0.));
#11596=DIRECTION('center_axis',(0.,1.,0.));
#11597=DIRECTION('ref_axis',(1.,0.,0.));
#11598=DIRECTION('center_axis',(0.,1.,0.));
#11599=DIRECTION('ref_axis',(1.,0.,0.));
#11600=DIRECTION('',(0.,1.,0.));
#11601=DIRECTION('center_axis',(0.,1.,0.));
#11602=DIRECTION('ref_axis',(1.,0.,0.));
#11603=DIRECTION('center_axis',(0.,1.,0.));
#11604=DIRECTION('ref_axis',(1.,0.,0.));
#11605=DIRECTION('',(0.,1.,0.));
#11606=DIRECTION('center_axis',(0.,1.,0.));
#11607=DIRECTION('ref_axis',(1.,0.,0.));
#11608=DIRECTION('center_axis',(0.,1.,0.));
#11609=DIRECTION('ref_axis',(1.,0.,0.));
#11610=DIRECTION('',(0.,1.,0.));
#11611=DIRECTION('center_axis',(0.,1.,0.));
#11612=DIRECTION('ref_axis',(1.,0.,0.));
#11613=DIRECTION('center_axis',(0.,1.,0.));
#11614=DIRECTION('ref_axis',(1.,0.,0.));
#11615=DIRECTION('',(0.,1.,0.));
#11616=DIRECTION('center_axis',(0.,1.,0.));
#11617=DIRECTION('ref_axis',(1.,0.,0.));
#11618=DIRECTION('center_axis',(0.,1.,0.));
#11619=DIRECTION('ref_axis',(1.,0.,0.));
#11620=DIRECTION('center_axis',(1.,0.,0.));
#11621=DIRECTION('ref_axis',(0.,1.,0.));
#11622=DIRECTION('',(0.,1.,0.));
#11623=DIRECTION('',(0.,1.,0.));
#11624=DIRECTION('',(0.,0.,1.));
#11625=DIRECTION('',(0.,1.,0.));
#11626=DIRECTION('center_axis',(0.,-1.,0.));
#11627=DIRECTION('ref_axis',(1.,0.,0.));
#11628=DIRECTION('',(1.,0.,0.));
#11629=DIRECTION('',(1.,0.,0.));
#11630=DIRECTION('center_axis',(0.,0.,1.));
#11631=DIRECTION('ref_axis',(1.,0.,0.));
#11632=DIRECTION('center_axis',(0.,0.,1.));
#11633=DIRECTION('ref_axis',(1.,0.,0.));
#14605=CARTESIAN_POINT('',(0.,0.,0.));
#14606=CARTESIAN_POINT('Origin',(-2.9,0.9,2.6));
#14607=CARTESIAN_POINT('',(-2.5,1.24003676271839,2.6));
#14608=CARTESIAN_POINT('',(-2.5,0.559963237281614,2.6));
#14609=CARTESIAN_POINT('',(-2.5,1.3,2.6));
#14610=CARTESIAN_POINT('Origin',(-2.9,0.9,2.6));
#14611=CARTESIAN_POINT('Origin',(-2.9,0.9,2.));
#14612=CARTESIAN_POINT('',(-2.5,1.24003676271839,2.));
#14613=CARTESIAN_POINT('',(-2.5,1.24003676271839,2.));
#14614=CARTESIAN_POINT('',(-2.5,0.559963237281614,2.));
#14615=CARTESIAN_POINT('Origin',(-2.9,0.9,2.));
#14616=CARTESIAN_POINT('',(-2.5,0.559963237281614,2.));
#14617=CARTESIAN_POINT('Origin',(2.9,0.9,2.));
#14618=CARTESIAN_POINT('',(2.5,1.24003676271839,2.6));
#14619=CARTESIAN_POINT('',(2.5,1.24003676271839,2.));
#14620=CARTESIAN_POINT('',(2.5,1.24003676271839,2.));
#14621=CARTESIAN_POINT('',(2.5,0.559963237281614,2.6));
#14622=CARTESIAN_POINT('Origin',(2.9,0.9,2.6));
#14623=CARTESIAN_POINT('',(2.5,0.559963237281614,2.));
#14624=CARTESIAN_POINT('',(2.5,0.559963237281614,2.));
#14625=CARTESIAN_POINT('Origin',(2.9,0.9,2.));
#14626=CARTESIAN_POINT('Origin',(2.9,0.9,2.6));
#14627=CARTESIAN_POINT('',(2.5,0.45,2.6));
#14628=CARTESIAN_POINT('Origin',(-2.5,1.7,2.));
#14629=CARTESIAN_POINT('',(-2.5,0.,2.));
#14630=CARTESIAN_POINT('',(-2.5,1.7,2.));
#14631=CARTESIAN_POINT('',(-2.5,0.,7.));
#14632=CARTESIAN_POINT('',(-2.5,0.,2.));
#14633=CARTESIAN_POINT('',(-2.5,1.7,7.));
#14634=CARTESIAN_POINT('',(-2.5,1.7,7.));
#14635=CARTESIAN_POINT('',(-2.5,1.7,2.));
#14636=CARTESIAN_POINT('',(-2.5,1.7,2.));
#14637=CARTESIAN_POINT('',(-2.5,1.7,2.));
#14638=CARTESIAN_POINT('Origin',(-1.2,0.6,1.9));
#14639=CARTESIAN_POINT('',(-1.41,0.6,2.));
#14640=CARTESIAN_POINT('Origin',(-1.2,0.6,2.));
#14641=CARTESIAN_POINT('',(-1.41,0.6,3.1));
#14642=CARTESIAN_POINT('',(-1.41,0.6,1.9));
#14643=CARTESIAN_POINT('Origin',(-1.2,0.6,3.1));
#14644=CARTESIAN_POINT('Origin',(-1.2,0.6,3.1));
#14645=CARTESIAN_POINT('Origin',(1.2,0.6,1.9));
#14646=CARTESIAN_POINT('',(0.99,0.6,2.));
#14647=CARTESIAN_POINT('Origin',(1.2,0.6,2.));
#14648=CARTESIAN_POINT('',(0.99,0.6,3.1));
#14649=CARTESIAN_POINT('',(0.99,0.6,1.9));
#14650=CARTESIAN_POINT('Origin',(1.2,0.6,3.1));
#14651=CARTESIAN_POINT('Origin',(1.2,0.6,3.1));
#14652=CARTESIAN_POINT('Origin',(0.,1.2,4.4));
#14653=CARTESIAN_POINT('',(0.2,1.2,5.73389626792531));
#14654=CARTESIAN_POINT('',(-0.2,1.2,5.73389626792531));
#14655=CARTESIAN_POINT('Ctrl Pts',(0.2,1.2,5.73389626792531));
#14656=CARTESIAN_POINT('Ctrl Pts',(0.2,1.22515924611223,5.73389626792531));
#14657=CARTESIAN_POINT('Ctrl Pts',(0.194963049432274,1.25196535332185,5.73474532770021));
#14658=CARTESIAN_POINT('Ctrl Pts',(0.1745390117426,1.30122807600043,5.73779753882153));
#14659=CARTESIAN_POINT('Ctrl Pts',(0.159154241644127,1.32368847083049,5.73995502329995));
#14660=CARTESIAN_POINT('Ctrl Pts',(0.123688872270436,1.35915384020418,5.74399340066366));
#14661=CARTESIAN_POINT('Ctrl Pts',(0.101228304743543,1.37453892520694,5.7461387706165));
#14662=CARTESIAN_POINT('Ctrl Pts',(0.0519649901302406,1.39496319170947,
5.74916317792714));
#14663=CARTESIAN_POINT('Ctrl Pts',(0.0251586765531237,1.4,5.75));
#14664=CARTESIAN_POINT('Ctrl Pts',(-0.0251586765531237,1.4,5.75));
#14665=CARTESIAN_POINT('Ctrl Pts',(-0.0519649901302405,1.39496319170947,
5.74916317792714));
#14666=CARTESIAN_POINT('Ctrl Pts',(-0.101228304743543,1.37453892520694,
5.7461387706165));
#14667=CARTESIAN_POINT('Ctrl Pts',(-0.123688872270436,1.35915384020418,
5.74399340066366));
#14668=CARTESIAN_POINT('Ctrl Pts',(-0.159154241644127,1.32368847083049,
5.73995502329995));
#14669=CARTESIAN_POINT('Ctrl Pts',(-0.1745390117426,1.30122807600043,5.73779753882153));
#14670=CARTESIAN_POINT('Ctrl Pts',(-0.194963049432274,1.25196535332185,
5.73474532770021));
#14671=CARTESIAN_POINT('Ctrl Pts',(-0.2,1.22515924611223,5.73389626792531));
#14672=CARTESIAN_POINT('Ctrl Pts',(-0.2,1.2,5.73389626792531));
#14673=CARTESIAN_POINT('',(0.2,1.2,5.06568542494924));
#14674=CARTESIAN_POINT('',(0.2,1.2,4.4));
#14675=CARTESIAN_POINT('',(-0.2,1.2,5.06568542494924));
#14676=CARTESIAN_POINT('Ctrl Pts',(-0.2,1.2,5.06568542494924));
#14677=CARTESIAN_POINT('Ctrl Pts',(-0.2,1.17467078791842,5.06568542494924));
#14678=CARTESIAN_POINT('Ctrl Pts',(-0.194898067853762,1.1477996053073,5.06756535657425));
#14679=CARTESIAN_POINT('Ctrl Pts',(-0.17443058152527,1.09858936400846,5.07418608255247));
#14680=CARTESIAN_POINT('Ctrl Pts',(-0.159074095999941,1.07623138352532,
5.0788137712126));
#14681=CARTESIAN_POINT('Ctrl Pts',(-0.123776803829002,1.04093409135438,
5.08737462203136));
#14682=CARTESIAN_POINT('Ctrl Pts',(-0.101415562391481,1.02557130277668,
5.09188739106068));
#14683=CARTESIAN_POINT('Ctrl Pts',(-0.0521932274441716,1.00509911583939,
5.09824047588691));
#14684=CARTESIAN_POINT('Ctrl Pts',(-0.0253174643734703,1.,5.1));
#14685=CARTESIAN_POINT('Ctrl Pts',(0.0253174643734703,1.,5.1));
#14686=CARTESIAN_POINT('Ctrl Pts',(0.0521932274441717,1.00509911583939,
5.09824047588691));
#14687=CARTESIAN_POINT('Ctrl Pts',(0.101415562391481,1.02557130277668,5.09188739106068));
#14688=CARTESIAN_POINT('Ctrl Pts',(0.123776803829002,1.04093409135438,5.08737462203136));
#14689=CARTESIAN_POINT('Ctrl Pts',(0.159074095999941,1.07623138352532,5.0788137712126));
#14690=CARTESIAN_POINT('Ctrl Pts',(0.17443058152527,1.09858936400846,5.07418608255247));
#14691=CARTESIAN_POINT('Ctrl Pts',(0.194898067853762,1.1477996053073,5.06756535657425));
#14692=CARTESIAN_POINT('Ctrl Pts',(0.2,1.17467078791842,5.06568542494924));
#14693=CARTESIAN_POINT('Ctrl Pts',(0.2,1.2,5.06568542494924));
#14694=CARTESIAN_POINT('',(-0.2,1.2,4.4));
#14695=CARTESIAN_POINT('',(-0.2,1.2,6.35));
#14696=CARTESIAN_POINT('',(-0.2,1.2,4.4));
#14697=CARTESIAN_POINT('Origin',(0.,1.2,6.35));
#14698=CARTESIAN_POINT('Origin',(0.,-0.1,4.5));
#14699=CARTESIAN_POINT('',(-0.6,0.,4.5));
#14700=CARTESIAN_POINT('Origin',(0.,0.,4.5));
#14701=CARTESIAN_POINT('',(-0.6,1.2,4.5));
#14702=CARTESIAN_POINT('',(-0.6,-0.1,4.5));
#14703=CARTESIAN_POINT('Origin',(0.,1.2,4.5));
#14704=CARTESIAN_POINT('Origin',(0.,1.2,4.5));
#14705=CARTESIAN_POINT('Origin',(0.,1.2,6.35));
#14706=CARTESIAN_POINT('',(-0.123389626792531,1.7,6.35));
#14707=CARTESIAN_POINT('',(0.123389626792531,1.7,6.35));
#14708=CARTESIAN_POINT('',(1.25,1.7,6.35));
#14709=CARTESIAN_POINT('Origin',(0.,1.2,6.35));
#14710=CARTESIAN_POINT('Origin',(0.,1.2,6.35));
#14711=CARTESIAN_POINT('',(-0.123389626792531,1.7,7.));
#14712=CARTESIAN_POINT('',(-0.123389626792531,1.7,6.35));
#14713=CARTESIAN_POINT('',(0.123389626792531,1.7,7.));
#14714=CARTESIAN_POINT('Origin',(0.,1.2,7.));
#14715=CARTESIAN_POINT('',(0.123389626792531,1.7,6.35));
#14716=CARTESIAN_POINT('Origin',(2.5,1.7,2.));
#14717=CARTESIAN_POINT('',(2.5,1.7,7.));
#14718=CARTESIAN_POINT('',(2.5,1.7,7.));
#14719=CARTESIAN_POINT('',(2.5,1.7,2.));
#14720=CARTESIAN_POINT('',(2.5,1.7,2.));
#14721=CARTESIAN_POINT('',(2.5,1.7,2.));
#14722=CARTESIAN_POINT('',(2.5,1.7,7.));
#14723=CARTESIAN_POINT('',(1.725,1.7,2.5));
#14724=CARTESIAN_POINT('Origin',(2.,1.7,2.5));
#14725=CARTESIAN_POINT('',(-2.275,1.7,6.5));
#14726=CARTESIAN_POINT('Origin',(-2.,1.7,6.5));
#14727=CARTESIAN_POINT('',(-2.275,1.7,2.5));
#14728=CARTESIAN_POINT('Origin',(-2.,1.7,2.5));
#14729=CARTESIAN_POINT('',(1.725,1.7,6.5));
#14730=CARTESIAN_POINT('Origin',(2.,1.7,6.5));
#14731=CARTESIAN_POINT('',(-1.25,1.7,4.5));
#14732=CARTESIAN_POINT('Origin',(0.,1.7,4.5));
#14733=CARTESIAN_POINT('Origin',(2.,-0.1,2.5));
#14734=CARTESIAN_POINT('',(1.725,0.,2.5));
#14735=CARTESIAN_POINT('Origin',(2.,0.,2.5));
#14736=CARTESIAN_POINT('',(1.725,-0.1,2.5));
#14737=CARTESIAN_POINT('Origin',(-2.,-0.1,6.5));
#14738=CARTESIAN_POINT('',(-2.275,0.,6.5));
#14739=CARTESIAN_POINT('Origin',(-2.,0.,6.5));
#14740=CARTESIAN_POINT('',(-2.275,-0.1,6.5));
#14741=CARTESIAN_POINT('Origin',(-2.,-0.1,2.5));
#14742=CARTESIAN_POINT('',(-2.275,0.,2.5));
#14743=CARTESIAN_POINT('Origin',(-2.,0.,2.5));
#14744=CARTESIAN_POINT('',(-2.275,-0.1,2.5));
#14745=CARTESIAN_POINT('Origin',(2.,-0.1,6.5));
#14746=CARTESIAN_POINT('',(1.725,0.,6.5));
#14747=CARTESIAN_POINT('Origin',(2.,0.,6.5));
#14748=CARTESIAN_POINT('',(1.725,-0.1,6.5));
#14749=CARTESIAN_POINT('Origin',(0.,1.2,4.5));
#14750=CARTESIAN_POINT('',(-1.25,1.2,4.5));
#14751=CARTESIAN_POINT('Origin',(0.,1.2,4.5));
#14752=CARTESIAN_POINT('',(-1.25,1.2,4.5));
#14753=CARTESIAN_POINT('Origin',(0.,1.2,4.5));
#14754=CARTESIAN_POINT('Origin',(0.,1.2,4.5));
#14755=CARTESIAN_POINT('Origin',(2.5,0.,2.));
#14756=CARTESIAN_POINT('',(2.5,0.,2.));
#14757=CARTESIAN_POINT('',(2.5,0.,7.));
#14758=CARTESIAN_POINT('',(2.5,0.,7.));
#14759=CARTESIAN_POINT('',(2.5,0.,2.));
#14760=CARTESIAN_POINT('',(2.5,0.,2.));
#14761=CARTESIAN_POINT('',(2.5,0.,2.));
#14762=CARTESIAN_POINT('Origin',(-2.5,0.,2.));
#14763=CARTESIAN_POINT('',(-2.5,0.,2.));
#14764=CARTESIAN_POINT('',(-2.5,0.,7.));
#14765=CARTESIAN_POINT('Origin',(0.,0.85,7.));
#14766=CARTESIAN_POINT('Origin',(0.,0.85,2.));
#18904=UNCERTAINTY_MEASURE_WITH_UNIT(LENGTH_MEASURE(0.001),#19044,
'DISTANCE_ACCURACY_VALUE',
'Maximum model space distance between geometric entities at asserted c
onnectivities');
#18972=UNCERTAINTY_MEASURE_WITH_UNIT(LENGTH_MEASURE(0.001),#19044,
'DISTANCE_ACCURACY_VALUE',
'Maximum model space distance between geometric entities at asserted c
onnectivities');
#18975=(
GEOMETRIC_REPRESENTATION_CONTEXT(3)
GLOBAL_UNCERTAINTY_ASSIGNED_CONTEXT((#18904))
GLOBAL_UNIT_ASSIGNED_CONTEXT((#19044,#19046,#19047))
REPRESENTATION_CONTEXT('','3D')
);
#19043=(
GEOMETRIC_REPRESENTATION_CONTEXT(3)
GLOBAL_UNCERTAINTY_ASSIGNED_CONTEXT((#18972))
GLOBAL_UNIT_ASSIGNED_CONTEXT((#19044,#19046,#19047))
REPRESENTATION_CONTEXT('','3D')
);
#19044=(
LENGTH_UNIT()
NAMED_UNIT(*)
SI_UNIT(.CENTI.,.METRE.)
);
#19046=(
NAMED_UNIT(*)
PLANE_ANGLE_UNIT()
SI_UNIT($,.RADIAN.)
);
#19047=(
NAMED_UNIT(*)
SI_UNIT($,.STERADIAN.)
SOLID_ANGLE_UNIT()
);
#19050=SHAPE_DEFINITION_REPRESENTATION(#19120,#19308);
#19120=PRODUCT_DEFINITION_SHAPE('',$,#19379);
#19308=SHAPE_REPRESENTATION('',(#10245),#18975);
#19376=PRODUCT_DEFINITION_CONTEXT('part definition',#19588,'design');
#19379=PRODUCT_DEFINITION('2026-11-03-00-38-46-435','Front cap',#19449,
#19376);
#19449=PRODUCT_DEFINITION_FORMATION('',$,#19592);
#19588=APPLICATION_CONTEXT(
'Core Data for Automotive Mechanical Design Process');
#19589=PRODUCT_CONTEXT('part definition',#19588,'mechanical');
#19592=PRODUCT('2026-11-03-00-38-46-435','Front cap','Front cap',(#19589));
#19661=PRESENTATION_STYLE_ASSIGNMENT((#19667));
#19667=SURFACE_STYLE_USAGE(.BOTH.,#19673);
#19673=SURFACE_SIDE_STYLE('',(#19679));
#19679=SURFACE_STYLE_FILL_AREA(#19685);
#19685=FILL_AREA_STYLE('CAD Library Painted - Engineering blue',(#19691));
#19691=FILL_AREA_STYLE_COLOUR('CAD Library Painted - Engineering blue',
#19697);
#19697=COLOUR_RGB('CAD Library Painted - Engineering blue',0.12156862745098,
0.356862745098039,0.6);
ENDSEC;
END-ISO-10303-21;
